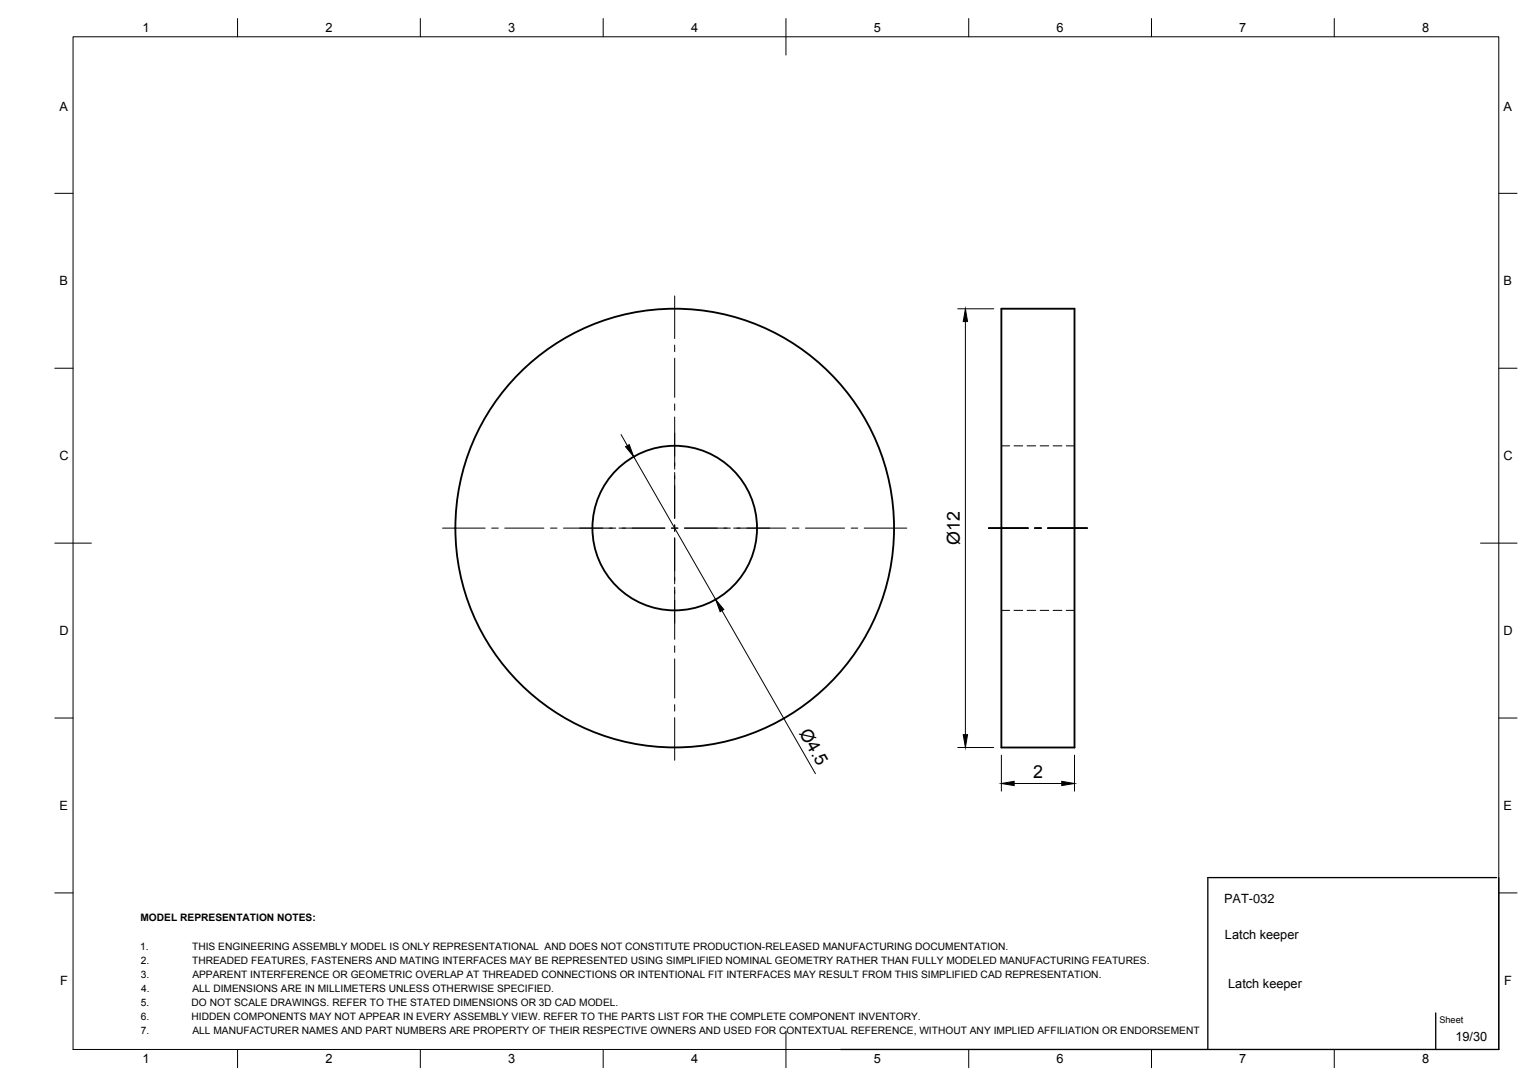
ISO-10303-21;
HEADER;
/* Generated by software containing ST-Developer
 * from STEP Tools, Inc. (www.steptools.com) 
 */

FILE_DESCRIPTION(
/* description */ ('Drill jig with bushing plate'),
/* implementation_level */ '2;1');

FILE_NAME(
/* name */ 'Latch keeper.step',
/* time_stamp */ '2026-10-27T10:51:08-07:00',
/* author */ (''),
/* organization */ (''),
/* preprocessor_version */ 'ST-DEVELOPER v20.2',
/* originating_system */ 'Autodesk Translation Framework v15.17.0.0',
/* authorisation */ '');

FILE_SCHEMA (('AUTOMOTIVE_DESIGN { 1 0 10303 214 3 1 1 }'));
ENDSEC;

DATA;
#10=MECHANICAL_DESIGN_GEOMETRIC_PRESENTATION_REPRESENTATION('',(#237),#6638);
#189=SHAPE_REPRESENTATION_RELATIONSHIP('SRR','None',#6753,#213);
#213=ADVANCED_BREP_SHAPE_REPRESENTATION('',(#261),#6626);
#237=STYLED_ITEM('',(#6936),#261);
#261=MANIFOLD_SOLID_BREP('Body1',#3604);
#341=FACE_BOUND('',#909,.T.);
#342=FACE_BOUND('',#911,.T.);
#440=PLANE('',#4129);
#441=PLANE('',#4130);
#620=FACE_OUTER_BOUND('',#906,.T.);
#621=FACE_OUTER_BOUND('',#907,.T.);
#622=FACE_OUTER_BOUND('',#908,.T.);
#623=FACE_OUTER_BOUND('',#910,.T.);
#906=EDGE_LOOP('',(#2927,#2928,#2929,#2930));
#907=EDGE_LOOP('',(#2931,#2932,#2933,#2934));
#908=EDGE_LOOP('',(#2935));
#909=EDGE_LOOP('',(#2936));
#910=EDGE_LOOP('',(#2937));
#911=EDGE_LOOP('',(#2938));
#1167=LINE('',#6133,#1428);
#1168=LINE('',#6139,#1429);
#1428=VECTOR('',#4954,0.225);
#1429=VECTOR('',#4961,0.6);
#1658=CIRCLE('',#4124,0.225);
#1659=CIRCLE('',#4125,0.225);
#1660=CIRCLE('',#4127,0.6);
#1661=CIRCLE('',#4128,0.6);
#1884=VERTEX_POINT('',#6130);
#1885=VERTEX_POINT('',#6132);
#1886=VERTEX_POINT('',#6136);
#1887=VERTEX_POINT('',#6138);
#2251=EDGE_CURVE('',#1884,#1884,#1658,.T.);
#2252=EDGE_CURVE('',#1884,#1885,#1167,.T.);
#2253=EDGE_CURVE('',#1885,#1885,#1659,.T.);
#2254=EDGE_CURVE('',#1886,#1886,#1660,.T.);
#2255=EDGE_CURVE('',#1886,#1887,#1168,.T.);
#2256=EDGE_CURVE('',#1887,#1887,#1661,.T.);
#2927=ORIENTED_EDGE('',*,*,#2251,.F.);
#2928=ORIENTED_EDGE('',*,*,#2252,.T.);
#2929=ORIENTED_EDGE('',*,*,#2253,.T.);
#2930=ORIENTED_EDGE('',*,*,#2252,.F.);
#2931=ORIENTED_EDGE('',*,*,#2254,.F.);
#2932=ORIENTED_EDGE('',*,*,#2255,.T.);
#2933=ORIENTED_EDGE('',*,*,#2256,.T.);
#2934=ORIENTED_EDGE('',*,*,#2255,.F.);
#2935=ORIENTED_EDGE('',*,*,#2254,.T.);
#2936=ORIENTED_EDGE('',*,*,#2251,.T.);
#2937=ORIENTED_EDGE('',*,*,#2256,.F.);
#2938=ORIENTED_EDGE('',*,*,#2253,.F.);
#3348=CYLINDRICAL_SURFACE('',#4123,0.225);
#3349=CYLINDRICAL_SURFACE('',#4126,0.6);
#3495=ADVANCED_FACE('',(#620),#3348,.F.);
#3496=ADVANCED_FACE('',(#621),#3349,.T.);
#3497=ADVANCED_FACE('',(#622,#341),#440,.T.);
#3498=ADVANCED_FACE('',(#623,#342),#441,.F.);
#3604=CLOSED_SHELL('',(#3495,#3496,#3497,#3498));
#4122=AXIS2_PLACEMENT_3D('',#6128,#4948,#4949);
#4123=AXIS2_PLACEMENT_3D('',#6129,#4950,#4951);
#4124=AXIS2_PLACEMENT_3D('',#6131,#4952,#4953);
#4125=AXIS2_PLACEMENT_3D('',#6134,#4955,#4956);
#4126=AXIS2_PLACEMENT_3D('',#6135,#4957,#4958);
#4127=AXIS2_PLACEMENT_3D('',#6137,#4959,#4960);
#4128=AXIS2_PLACEMENT_3D('',#6140,#4962,#4963);
#4129=AXIS2_PLACEMENT_3D('',#6141,#4964,#4965);
#4130=AXIS2_PLACEMENT_3D('',#6142,#4966,#4967);
#4948=DIRECTION('axis',(0.,0.,1.));
#4949=DIRECTION('refdir',(1.,0.,0.));
#4950=DIRECTION('center_axis',(0.,0.,1.));
#4951=DIRECTION('ref_axis',(1.,0.,0.));
#4952=DIRECTION('center_axis',(0.,0.,-1.));
#4953=DIRECTION('ref_axis',(1.,0.,0.));
#4954=DIRECTION('',(0.,0.,-1.));
#4955=DIRECTION('center_axis',(0.,0.,-1.));
#4956=DIRECTION('ref_axis',(1.,0.,0.));
#4957=DIRECTION('center_axis',(0.,0.,1.));
#4958=DIRECTION('ref_axis',(1.,0.,0.));
#4959=DIRECTION('center_axis',(0.,0.,1.));
#4960=DIRECTION('ref_axis',(1.,0.,0.));
#4961=DIRECTION('',(0.,0.,-1.));
#4962=DIRECTION('center_axis',(0.,0.,1.));
#4963=DIRECTION('ref_axis',(1.,0.,0.));
#4964=DIRECTION('center_axis',(0.,0.,1.));
#4965=DIRECTION('ref_axis',(1.,0.,0.));
#4966=DIRECTION('center_axis',(0.,0.,1.));
#4967=DIRECTION('ref_axis',(1.,0.,0.));
#6128=CARTESIAN_POINT('',(0.,0.,0.));
#6129=CARTESIAN_POINT('Origin',(9.2,3.5,5.));
#6130=CARTESIAN_POINT('',(8.975,3.5,5.2));
#6131=CARTESIAN_POINT('Origin',(9.2,3.5,5.2));
#6132=CARTESIAN_POINT('',(8.975,3.5,5.));
#6133=CARTESIAN_POINT('',(8.975,3.5,5.));
#6134=CARTESIAN_POINT('Origin',(9.2,3.5,5.));
#6135=CARTESIAN_POINT('Origin',(9.2,3.5,5.));
#6136=CARTESIAN_POINT('',(8.6,3.5,5.2));
#6137=CARTESIAN_POINT('Origin',(9.2,3.5,5.2));
#6138=CARTESIAN_POINT('',(8.6,3.5,5.));
#6139=CARTESIAN_POINT('',(8.6,3.5,5.));
#6140=CARTESIAN_POINT('Origin',(9.2,3.5,5.));
#6141=CARTESIAN_POINT('Origin',(9.2,3.5,5.2));
#6142=CARTESIAN_POINT('Origin',(9.2,3.5,5.));
#6597=UNCERTAINTY_MEASURE_WITH_UNIT(LENGTH_MEASURE(0.001),#6639,
'DISTANCE_ACCURACY_VALUE',
'Maximum model space distance between geometric entities at asserted c
onnectivities');
#6609=UNCERTAINTY_MEASURE_WITH_UNIT(LENGTH_MEASURE(0.001),#6639,
'DISTANCE_ACCURACY_VALUE',
'Maximum model space distance between geometric entities at asserted c
onnectivities');
#6626=(
GEOMETRIC_REPRESENTATION_CONTEXT(3)
GLOBAL_UNCERTAINTY_ASSIGNED_CONTEXT((#6597))
GLOBAL_UNIT_ASSIGNED_CONTEXT((#6639,#6641,#6642))
REPRESENTATION_CONTEXT('','3D')
);
#6638=(
GEOMETRIC_REPRESENTATION_CONTEXT(3)
GLOBAL_UNCERTAINTY_ASSIGNED_CONTEXT((#6609))
GLOBAL_UNIT_ASSIGNED_CONTEXT((#6639,#6641,#6642))
REPRESENTATION_CONTEXT('','3D')
);
#6639=(
LENGTH_UNIT()
NAMED_UNIT(*)
SI_UNIT(.CENTI.,.METRE.)
);
#6641=(
NAMED_UNIT(*)
PLANE_ANGLE_UNIT()
SI_UNIT($,.RADIAN.)
);
#6642=(
NAMED_UNIT(*)
SI_UNIT($,.STERADIAN.)
SOLID_ANGLE_UNIT()
);
#6659=SHAPE_DEFINITION_REPRESENTATION(#6687,#6753);
#6687=PRODUCT_DEFINITION_SHAPE('',$,#6782);
#6753=SHAPE_REPRESENTATION('',(#4122),#6626);
#6765=PRODUCT_DEFINITION_CONTEXT('part definition',#6851,'design');
#6782=PRODUCT_DEFINITION('Latch keeper','Latch keeper',#6810,#6765);
#6810=PRODUCT_DEFINITION_FORMATION('',$,#6869);
#6851=APPLICATION_CONTEXT(
'Core Data for Automotive Mechanical Design Process');
#6852=PRODUCT_CONTEXT('part definition',#6851,'mechanical');
#6869=PRODUCT('Latch keeper','Latch keeper','Latch keeper',(#6852));
#6930=COLOUR_RGB('Sky Blue',0.24,0.69,0.87);
#6931=FILL_AREA_STYLE_COLOUR('',#6930);
#6932=FILL_AREA_STYLE('',(#6931));
#6933=SURFACE_STYLE_FILL_AREA(#6932);
#6934=SURFACE_SIDE_STYLE('',(#6933));
#6935=SURFACE_STYLE_USAGE(.BOTH.,#6934);
#6936=PRESENTATION_STYLE_ASSIGNMENT((#6935));
ENDSEC;
END-ISO-10303-21;
